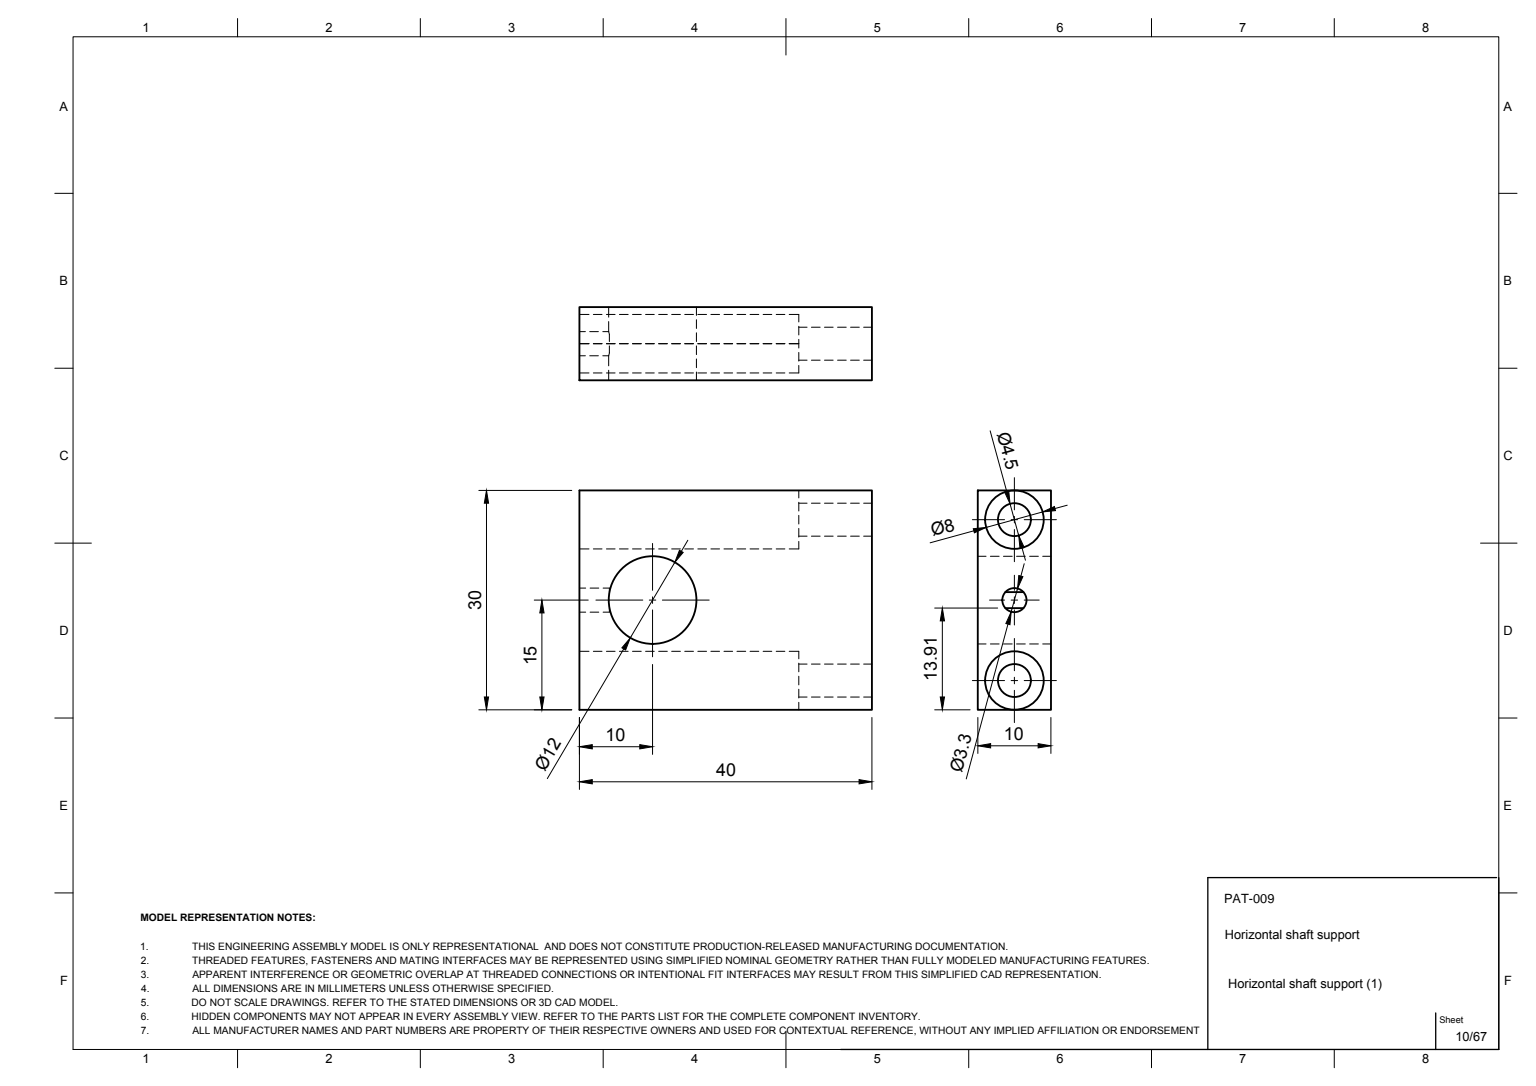
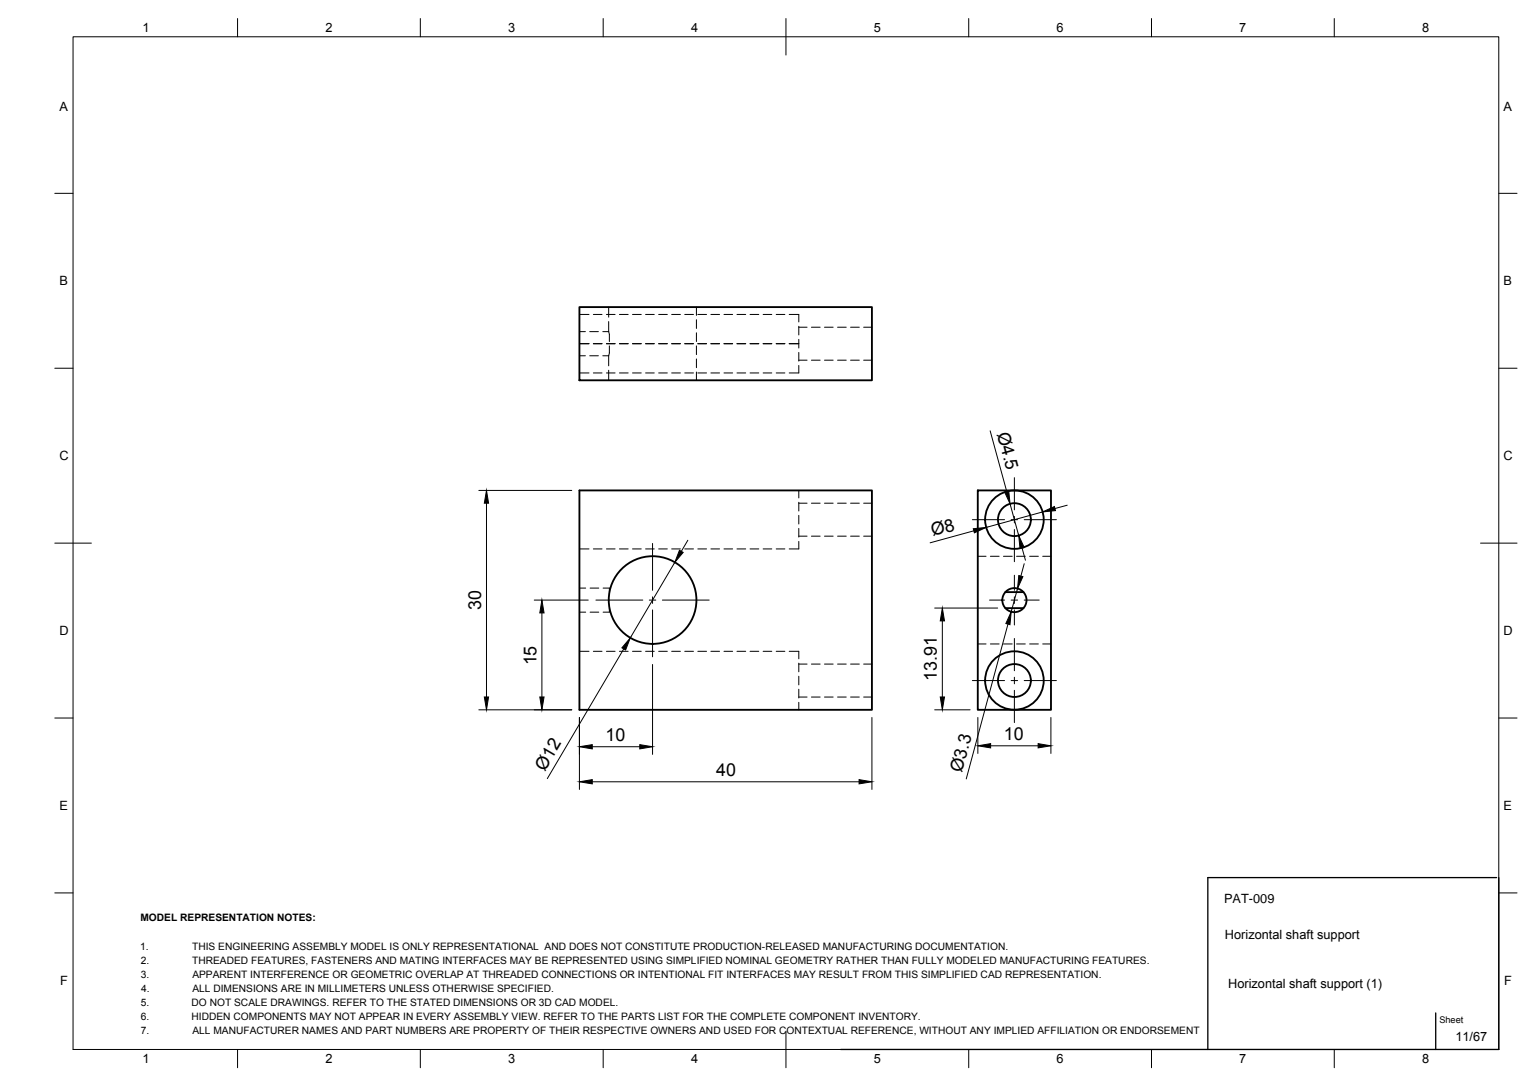
ISO-10303-21;
HEADER;
/* Generated by software containing ST-Developer
 * from STEP Tools, Inc. (www.steptools.com) 
 */

FILE_DESCRIPTION(
/* description */ ('Bell-crank linkage with push rods'),
/* implementation_level */ '2;1');

FILE_NAME(
/* name */ 'Horizontal shaft support (1).step',
/* time_stamp */ '2026-10-28T03:25:15-07:00',
/* author */ (''),
/* organization */ (''),
/* preprocessor_version */ 'ST-DEVELOPER v20.2',
/* originating_system */ 'Autodesk Translation Framework v15.17.0.0',
/* authorisation */ '');

FILE_SCHEMA (('AUTOMOTIVE_DESIGN { 1 0 10303 214 3 1 1 }'));
ENDSEC;

DATA;
#10=MECHANICAL_DESIGN_GEOMETRIC_PRESENTATION_REPRESENTATION('',(#610),#16678);
#465=B_SPLINE_CURVE_WITH_KNOTS('',3,(#14110,#14111,#14112,#14113,#14114,
#14115),.UNSPECIFIED.,.F.,.F.,(4,2,4),(0.635430324955932,0.687528937234027,
0.750024497760672),.UNSPECIFIED.);
#466=B_SPLINE_CURVE_WITH_KNOTS('',3,(#14119,#14120,#14121,#14122,#14123,
#14124),.UNSPECIFIED.,.F.,.F.,(4,2,4),(0.250008165920224,0.312503726446869,
0.364602338724963),.UNSPECIFIED.);
#467=B_SPLINE_CURVE_WITH_KNOTS('',3,(#14125,#14126,#14127,#14128,#14129,
#14130),.UNSPECIFIED.,.F.,.F.,(4,2,4),(0.135413993115483,0.187512605393579,
0.250008165920224),.UNSPECIFIED.);
#468=B_SPLINE_CURVE_WITH_KNOTS('',3,(#14131,#14132,#14133,#14134,#14135,
#14136),.UNSPECIFIED.,.F.,.F.,(4,2,4),(0.750024497760672,0.812520058287317,
0.864618670565412),.UNSPECIFIED.);
#502=SHAPE_REPRESENTATION_RELATIONSHIP('SRR','None',#16918,#556);
#556=ADVANCED_BREP_SHAPE_REPRESENTATION('',(#672),#16623);
#610=STYLED_ITEM('',(#17291),#672);
#672=MANIFOLD_SOLID_BREP('Body1',#8800);
#789=FACE_BOUND('',#1935,.T.);
#790=FACE_BOUND('',#1938,.T.);
#791=FACE_BOUND('',#1940,.T.);
#792=FACE_BOUND('',#1946,.T.);
#793=FACE_BOUND('',#1949,.T.);
#794=FACE_BOUND('',#1951,.T.);
#795=FACE_BOUND('',#1952,.T.);
#1013=PLANE('',#9667);
#1014=PLANE('',#9672);
#1015=PLANE('',#9676);
#1016=PLANE('',#9681);
#1017=PLANE('',#9683);
#1018=PLANE('',#9691);
#1019=PLANE('',#9692);
#1020=PLANE('',#9693);
#1021=PLANE('',#9694);
#1022=PLANE('',#9695);
#1342=FACE_OUTER_BOUND('',#1928,.T.);
#1343=FACE_OUTER_BOUND('',#1929,.T.);
#1344=FACE_OUTER_BOUND('',#1930,.T.);
#1345=FACE_OUTER_BOUND('',#1931,.T.);
#1346=FACE_OUTER_BOUND('',#1932,.T.);
#1347=FACE_OUTER_BOUND('',#1933,.T.);
#1348=FACE_OUTER_BOUND('',#1934,.T.);
#1349=FACE_OUTER_BOUND('',#1936,.T.);
#1350=FACE_OUTER_BOUND('',#1937,.T.);
#1351=FACE_OUTER_BOUND('',#1939,.T.);
#1352=FACE_OUTER_BOUND('',#1941,.T.);
#1353=FACE_OUTER_BOUND('',#1942,.T.);
#1354=FACE_OUTER_BOUND('',#1943,.T.);
#1355=FACE_OUTER_BOUND('',#1944,.T.);
#1356=FACE_OUTER_BOUND('',#1945,.T.);
#1357=FACE_OUTER_BOUND('',#1947,.T.);
#1358=FACE_OUTER_BOUND('',#1948,.T.);
#1359=FACE_OUTER_BOUND('',#1950,.T.);
#1928=EDGE_LOOP('',(#6347,#6348,#6349,#6350));
#1929=EDGE_LOOP('',(#6351,#6352,#6353,#6354));
#1930=EDGE_LOOP('',(#6355,#6356));
#1931=EDGE_LOOP('',(#6357,#6358,#6359,#6360,#6361,#6362,#6363,#6364,#6365));
#1932=EDGE_LOOP('',(#6366,#6367));
#1933=EDGE_LOOP('',(#6368,#6369,#6370,#6371));
#1934=EDGE_LOOP('',(#6372,#6373));
#1935=EDGE_LOOP('',(#6374));
#1936=EDGE_LOOP('',(#6375,#6376,#6377,#6378));
#1937=EDGE_LOOP('',(#6379,#6380));
#1938=EDGE_LOOP('',(#6381));
#1939=EDGE_LOOP('',(#6382,#6383,#6384,#6385,#6386,#6387,#6388,#6389,#6390,
#6391));
#1940=EDGE_LOOP('',(#6392));
#1941=EDGE_LOOP('',(#6393,#6394,#6395,#6396));
#1942=EDGE_LOOP('',(#6397,#6398,#6399,#6400));
#1943=EDGE_LOOP('',(#6401,#6402,#6403,#6404,#6405,#6406,#6407,#6408,#6409,
#6410,#6411,#6412));
#1944=EDGE_LOOP('',(#6413,#6414,#6415,#6416,#6417,#6418,#6419));
#1945=EDGE_LOOP('',(#6420,#6421,#6422,#6423));
#1946=EDGE_LOOP('',(#6424));
#1947=EDGE_LOOP('',(#6425,#6426,#6427,#6428,#6429,#6430,#6431));
#1948=EDGE_LOOP('',(#6432,#6433,#6434,#6435));
#1949=EDGE_LOOP('',(#6436));
#1950=EDGE_LOOP('',(#6437,#6438,#6439,#6440));
#1951=EDGE_LOOP('',(#6441));
#1952=EDGE_LOOP('',(#6442));
#2639=LINE('',#14087,#3188);
#2640=LINE('',#14091,#3189);
#2641=LINE('',#14096,#3190);
#2642=LINE('',#14100,#3191);
#2643=LINE('',#14105,#3192);
#2644=LINE('',#14138,#3193);
#2645=LINE('',#14141,#3194);
#2646=LINE('',#14144,#3195);
#2647=LINE('',#14151,#3196);
#2648=LINE('',#14159,#3197);
#2649=LINE('',#14160,#3198);
#2650=LINE('',#14162,#3199);
#2651=LINE('',#14164,#3200);
#2652=LINE('',#14165,#3201);
#2653=LINE('',#14166,#3202);
#2654=LINE('',#14170,#3203);
#2655=LINE('',#14174,#3204);
#2656=LINE('',#14178,#3205);
#2657=LINE('',#14180,#3206);
#2658=LINE('',#14185,#3207);
#2659=LINE('',#14186,#3208);
#2660=LINE('',#14187,#3209);
#2661=LINE('',#14190,#3210);
#2662=LINE('',#14191,#3211);
#2663=LINE('',#14194,#3212);
#2664=LINE('',#14195,#3213);
#2665=LINE('',#14197,#3214);
#3188=VECTOR('',#11153,0.4);
#3189=VECTOR('',#11156,1.);
#3190=VECTOR('',#11161,0.4);
#3191=VECTOR('',#11164,1.);
#3192=VECTOR('',#11169,1.);
#3193=VECTOR('',#11176,0.164999999999999);
#3194=VECTOR('',#11181,1.);
#3195=VECTOR('',#11186,1.);
#3196=VECTOR('',#11197,1.);
#3197=VECTOR('',#11206,1.);
#3198=VECTOR('',#11207,1.);
#3199=VECTOR('',#11208,1.);
#3200=VECTOR('',#11209,1.);
#3201=VECTOR('',#11210,1.);
#3202=VECTOR('',#11211,1.);
#3203=VECTOR('',#11216,0.225);
#3204=VECTOR('',#11221,0.225);
#3205=VECTOR('',#11226,0.6);
#3206=VECTOR('',#11227,0.6);
#3207=VECTOR('',#11232,1.);
#3208=VECTOR('',#11233,1.);
#3209=VECTOR('',#11234,1.);
#3210=VECTOR('',#11237,1.);
#3211=VECTOR('',#11238,1.);
#3212=VECTOR('',#11241,1.);
#3213=VECTOR('',#11242,1.);
#3214=VECTOR('',#11245,1.);
#3733=CIRCLE('',#9662,0.4);
#3734=CIRCLE('',#9663,0.4);
#3735=CIRCLE('',#9665,0.4);
#3736=CIRCLE('',#9666,0.4);
#3737=CIRCLE('',#9668,0.164999999999999);
#3738=CIRCLE('',#9670,0.164999999999999);
#3739=CIRCLE('',#9671,0.164999999999999);
#3740=CIRCLE('',#9674,0.4);
#3741=CIRCLE('',#9675,0.4);
#3742=CIRCLE('',#9677,0.225);
#3743=CIRCLE('',#9679,0.4);
#3744=CIRCLE('',#9680,0.4);
#3745=CIRCLE('',#9682,0.225);
#3746=CIRCLE('',#9685,0.225);
#3747=CIRCLE('',#9687,0.225);
#3748=CIRCLE('',#9689,0.6);
#3749=CIRCLE('',#9690,0.6);
#4263=VERTEX_POINT('',#14085);
#4264=VERTEX_POINT('',#14086);
#4265=VERTEX_POINT('',#14088);
#4266=VERTEX_POINT('',#14090);
#4267=VERTEX_POINT('',#14094);
#4268=VERTEX_POINT('',#14095);
#4269=VERTEX_POINT('',#14097);
#4270=VERTEX_POINT('',#14099);
#4271=VERTEX_POINT('',#14103);
#4272=VERTEX_POINT('',#14104);
#4273=VERTEX_POINT('',#14108);
#4274=VERTEX_POINT('',#14109);
#4275=VERTEX_POINT('',#14116);
#4276=VERTEX_POINT('',#14118);
#4277=VERTEX_POINT('',#14137);
#4278=VERTEX_POINT('',#14147);
#4279=VERTEX_POINT('',#14154);
#4280=VERTEX_POINT('',#14157);
#4281=VERTEX_POINT('',#14158);
#4282=VERTEX_POINT('',#14161);
#4283=VERTEX_POINT('',#14163);
#4284=VERTEX_POINT('',#14168);
#4285=VERTEX_POINT('',#14172);
#4286=VERTEX_POINT('',#14176);
#4287=VERTEX_POINT('',#14179);
#4288=VERTEX_POINT('',#14183);
#4289=VERTEX_POINT('',#14184);
#4290=VERTEX_POINT('',#14189);
#4291=VERTEX_POINT('',#14193);
#5051=EDGE_CURVE('',#4263,#4264,#2639,.T.);
#5052=EDGE_CURVE('',#4265,#4263,#3733,.T.);
#5053=EDGE_CURVE('',#4265,#4266,#2640,.T.);
#5054=EDGE_CURVE('',#4264,#4266,#3734,.T.);
#5055=EDGE_CURVE('',#4267,#4268,#2641,.T.);
#5056=EDGE_CURVE('',#4269,#4267,#3735,.T.);
#5057=EDGE_CURVE('',#4269,#4270,#2642,.T.);
#5058=EDGE_CURVE('',#4268,#4270,#3736,.T.);
#5059=EDGE_CURVE('',#4271,#4272,#2643,.T.);
#5060=EDGE_CURVE('',#4271,#4272,#3737,.T.);
#5061=EDGE_CURVE('',#4273,#4274,#465,.T.);
#5062=EDGE_CURVE('',#4275,#4273,#3738,.T.);
#5063=EDGE_CURVE('',#4276,#4275,#466,.T.);
#5064=EDGE_CURVE('',#4272,#4276,#467,.T.);
#5065=EDGE_CURVE('',#4274,#4271,#468,.T.);
#5066=EDGE_CURVE('',#4274,#4277,#2644,.T.);
#5067=EDGE_CURVE('',#4277,#4277,#3739,.T.);
#5068=EDGE_CURVE('',#4275,#4273,#2645,.T.);
#5069=EDGE_CURVE('',#4270,#4268,#3740,.T.);
#5070=EDGE_CURVE('',#4269,#4270,#2646,.T.);
#5071=EDGE_CURVE('',#4267,#4269,#3741,.T.);
#5072=EDGE_CURVE('',#4278,#4278,#3742,.T.);
#5073=EDGE_CURVE('',#4266,#4264,#3743,.T.);
#5074=EDGE_CURVE('',#4265,#4266,#2647,.T.);
#5075=EDGE_CURVE('',#4263,#4265,#3744,.T.);
#5076=EDGE_CURVE('',#4279,#4279,#3745,.T.);
#5077=EDGE_CURVE('',#4280,#4281,#2648,.T.);
#5078=EDGE_CURVE('',#4281,#4270,#2649,.T.);
#5079=EDGE_CURVE('',#4270,#4282,#2650,.T.);
#5080=EDGE_CURVE('',#4282,#4283,#2651,.T.);
#5081=EDGE_CURVE('',#4283,#4266,#2652,.T.);
#5082=EDGE_CURVE('',#4266,#4280,#2653,.T.);
#5083=EDGE_CURVE('',#4284,#4284,#3746,.T.);
#5084=EDGE_CURVE('',#4284,#4278,#2654,.T.);
#5085=EDGE_CURVE('',#4285,#4285,#3747,.T.);
#5086=EDGE_CURVE('',#4285,#4279,#2655,.T.);
#5087=EDGE_CURVE('',#4286,#4286,#3748,.T.);
#5088=EDGE_CURVE('',#4286,#4274,#2656,.T.);
#5089=EDGE_CURVE('',#4276,#4287,#2657,.T.);
#5090=EDGE_CURVE('',#4287,#4287,#3749,.T.);
#5091=EDGE_CURVE('',#4288,#4289,#2658,.T.);
#5092=EDGE_CURVE('',#4289,#4280,#2659,.T.);
#5093=EDGE_CURVE('',#4288,#4283,#2660,.T.);
#5094=EDGE_CURVE('',#4290,#4288,#2661,.T.);
#5095=EDGE_CURVE('',#4290,#4282,#2662,.T.);
#5096=EDGE_CURVE('',#4291,#4290,#2663,.T.);
#5097=EDGE_CURVE('',#4291,#4281,#2664,.T.);
#5098=EDGE_CURVE('',#4289,#4291,#2665,.T.);
#6347=ORIENTED_EDGE('',*,*,#5051,.F.);
#6348=ORIENTED_EDGE('',*,*,#5052,.F.);
#6349=ORIENTED_EDGE('',*,*,#5053,.T.);
#6350=ORIENTED_EDGE('',*,*,#5054,.F.);
#6351=ORIENTED_EDGE('',*,*,#5055,.F.);
#6352=ORIENTED_EDGE('',*,*,#5056,.F.);
#6353=ORIENTED_EDGE('',*,*,#5057,.T.);
#6354=ORIENTED_EDGE('',*,*,#5058,.F.);
#6355=ORIENTED_EDGE('',*,*,#5059,.F.);
#6356=ORIENTED_EDGE('',*,*,#5060,.T.);
#6357=ORIENTED_EDGE('',*,*,#5061,.F.);
#6358=ORIENTED_EDGE('',*,*,#5062,.F.);
#6359=ORIENTED_EDGE('',*,*,#5063,.F.);
#6360=ORIENTED_EDGE('',*,*,#5064,.F.);
#6361=ORIENTED_EDGE('',*,*,#5060,.F.);
#6362=ORIENTED_EDGE('',*,*,#5065,.F.);
#6363=ORIENTED_EDGE('',*,*,#5066,.T.);
#6364=ORIENTED_EDGE('',*,*,#5067,.F.);
#6365=ORIENTED_EDGE('',*,*,#5066,.F.);
#6366=ORIENTED_EDGE('',*,*,#5068,.F.);
#6367=ORIENTED_EDGE('',*,*,#5062,.T.);
#6368=ORIENTED_EDGE('',*,*,#5055,.T.);
#6369=ORIENTED_EDGE('',*,*,#5069,.F.);
#6370=ORIENTED_EDGE('',*,*,#5070,.F.);
#6371=ORIENTED_EDGE('',*,*,#5071,.F.);
#6372=ORIENTED_EDGE('',*,*,#5056,.T.);
#6373=ORIENTED_EDGE('',*,*,#5071,.T.);
#6374=ORIENTED_EDGE('',*,*,#5072,.F.);
#6375=ORIENTED_EDGE('',*,*,#5051,.T.);
#6376=ORIENTED_EDGE('',*,*,#5073,.F.);
#6377=ORIENTED_EDGE('',*,*,#5074,.F.);
#6378=ORIENTED_EDGE('',*,*,#5075,.F.);
#6379=ORIENTED_EDGE('',*,*,#5052,.T.);
#6380=ORIENTED_EDGE('',*,*,#5075,.T.);
#6381=ORIENTED_EDGE('',*,*,#5076,.F.);
#6382=ORIENTED_EDGE('',*,*,#5077,.T.);
#6383=ORIENTED_EDGE('',*,*,#5078,.T.);
#6384=ORIENTED_EDGE('',*,*,#5069,.T.);
#6385=ORIENTED_EDGE('',*,*,#5058,.T.);
#6386=ORIENTED_EDGE('',*,*,#5079,.T.);
#6387=ORIENTED_EDGE('',*,*,#5080,.T.);
#6388=ORIENTED_EDGE('',*,*,#5081,.T.);
#6389=ORIENTED_EDGE('',*,*,#5073,.T.);
#6390=ORIENTED_EDGE('',*,*,#5054,.T.);
#6391=ORIENTED_EDGE('',*,*,#5082,.T.);
#6392=ORIENTED_EDGE('',*,*,#5067,.T.);
#6393=ORIENTED_EDGE('',*,*,#5083,.F.);
#6394=ORIENTED_EDGE('',*,*,#5084,.T.);
#6395=ORIENTED_EDGE('',*,*,#5072,.T.);
#6396=ORIENTED_EDGE('',*,*,#5084,.F.);
#6397=ORIENTED_EDGE('',*,*,#5085,.F.);
#6398=ORIENTED_EDGE('',*,*,#5086,.T.);
#6399=ORIENTED_EDGE('',*,*,#5076,.T.);
#6400=ORIENTED_EDGE('',*,*,#5086,.F.);
#6401=ORIENTED_EDGE('',*,*,#5087,.F.);
#6402=ORIENTED_EDGE('',*,*,#5088,.T.);
#6403=ORIENTED_EDGE('',*,*,#5065,.T.);
#6404=ORIENTED_EDGE('',*,*,#5059,.T.);
#6405=ORIENTED_EDGE('',*,*,#5064,.T.);
#6406=ORIENTED_EDGE('',*,*,#5089,.T.);
#6407=ORIENTED_EDGE('',*,*,#5090,.F.);
#6408=ORIENTED_EDGE('',*,*,#5089,.F.);
#6409=ORIENTED_EDGE('',*,*,#5063,.T.);
#6410=ORIENTED_EDGE('',*,*,#5068,.T.);
#6411=ORIENTED_EDGE('',*,*,#5061,.T.);
#6412=ORIENTED_EDGE('',*,*,#5088,.F.);
#6413=ORIENTED_EDGE('',*,*,#5091,.T.);
#6414=ORIENTED_EDGE('',*,*,#5092,.T.);
#6415=ORIENTED_EDGE('',*,*,#5082,.F.);
#6416=ORIENTED_EDGE('',*,*,#5053,.F.);
#6417=ORIENTED_EDGE('',*,*,#5074,.T.);
#6418=ORIENTED_EDGE('',*,*,#5081,.F.);
#6419=ORIENTED_EDGE('',*,*,#5093,.F.);
#6420=ORIENTED_EDGE('',*,*,#5094,.T.);
#6421=ORIENTED_EDGE('',*,*,#5093,.T.);
#6422=ORIENTED_EDGE('',*,*,#5080,.F.);
#6423=ORIENTED_EDGE('',*,*,#5095,.F.);
#6424=ORIENTED_EDGE('',*,*,#5090,.T.);
#6425=ORIENTED_EDGE('',*,*,#5096,.T.);
#6426=ORIENTED_EDGE('',*,*,#5095,.T.);
#6427=ORIENTED_EDGE('',*,*,#5079,.F.);
#6428=ORIENTED_EDGE('',*,*,#5057,.F.);
#6429=ORIENTED_EDGE('',*,*,#5070,.T.);
#6430=ORIENTED_EDGE('',*,*,#5078,.F.);
#6431=ORIENTED_EDGE('',*,*,#5097,.F.);
#6432=ORIENTED_EDGE('',*,*,#5098,.T.);
#6433=ORIENTED_EDGE('',*,*,#5097,.T.);
#6434=ORIENTED_EDGE('',*,*,#5077,.F.);
#6435=ORIENTED_EDGE('',*,*,#5092,.F.);
#6436=ORIENTED_EDGE('',*,*,#5087,.T.);
#6437=ORIENTED_EDGE('',*,*,#5098,.F.);
#6438=ORIENTED_EDGE('',*,*,#5091,.F.);
#6439=ORIENTED_EDGE('',*,*,#5094,.F.);
#6440=ORIENTED_EDGE('',*,*,#5096,.F.);
#6441=ORIENTED_EDGE('',*,*,#5083,.T.);
#6442=ORIENTED_EDGE('',*,*,#5085,.T.);
#8115=CYLINDRICAL_SURFACE('',#9661,0.4);
#8116=CYLINDRICAL_SURFACE('',#9664,0.4);
#8117=CYLINDRICAL_SURFACE('',#9669,0.164999999999999);
#8118=CYLINDRICAL_SURFACE('',#9673,0.4);
#8119=CYLINDRICAL_SURFACE('',#9678,0.4);
#8120=CYLINDRICAL_SURFACE('',#9684,0.225);
#8121=CYLINDRICAL_SURFACE('',#9686,0.225);
#8122=CYLINDRICAL_SURFACE('',#9688,0.6);
#8367=ADVANCED_FACE('',(#1342),#8115,.F.);
#8368=ADVANCED_FACE('',(#1343),#8116,.F.);
#8369=ADVANCED_FACE('',(#1344),#1013,.T.);
#8370=ADVANCED_FACE('',(#1345),#8117,.F.);
#8371=ADVANCED_FACE('',(#1346),#1014,.T.);
#8372=ADVANCED_FACE('',(#1347),#8118,.F.);
#8373=ADVANCED_FACE('',(#1348,#789),#1015,.T.);
#8374=ADVANCED_FACE('',(#1349),#8119,.F.);
#8375=ADVANCED_FACE('',(#1350,#790),#1016,.T.);
#8376=ADVANCED_FACE('',(#1351,#791),#1017,.T.);
#8377=ADVANCED_FACE('',(#1352),#8120,.F.);
#8378=ADVANCED_FACE('',(#1353),#8121,.F.);
#8379=ADVANCED_FACE('',(#1354),#8122,.F.);
#8380=ADVANCED_FACE('',(#1355),#1018,.T.);
#8381=ADVANCED_FACE('',(#1356,#792),#1019,.T.);
#8382=ADVANCED_FACE('',(#1357),#1020,.T.);
#8383=ADVANCED_FACE('',(#1358,#793),#1021,.T.);
#8384=ADVANCED_FACE('',(#1359,#794,#795),#1022,.F.);
#8800=CLOSED_SHELL('',(#8367,#8368,#8369,#8370,#8371,#8372,#8373,#8374,
#8375,#8376,#8377,#8378,#8379,#8380,#8381,#8382,#8383,#8384));
#9660=AXIS2_PLACEMENT_3D('',#14083,#11149,#11150);
#9661=AXIS2_PLACEMENT_3D('',#14084,#11151,#11152);
#9662=AXIS2_PLACEMENT_3D('',#14089,#11154,#11155);
#9663=AXIS2_PLACEMENT_3D('',#14092,#11157,#11158);
#9664=AXIS2_PLACEMENT_3D('',#14093,#11159,#11160);
#9665=AXIS2_PLACEMENT_3D('',#14098,#11162,#11163);
#9666=AXIS2_PLACEMENT_3D('',#14101,#11165,#11166);
#9667=AXIS2_PLACEMENT_3D('',#14102,#11167,#11168);
#9668=AXIS2_PLACEMENT_3D('',#14106,#11170,#11171);
#9669=AXIS2_PLACEMENT_3D('',#14107,#11172,#11173);
#9670=AXIS2_PLACEMENT_3D('',#14117,#11174,#11175);
#9671=AXIS2_PLACEMENT_3D('',#14139,#11177,#11178);
#9672=AXIS2_PLACEMENT_3D('',#14140,#11179,#11180);
#9673=AXIS2_PLACEMENT_3D('',#14142,#11182,#11183);
#9674=AXIS2_PLACEMENT_3D('',#14143,#11184,#11185);
#9675=AXIS2_PLACEMENT_3D('',#14145,#11187,#11188);
#9676=AXIS2_PLACEMENT_3D('',#14146,#11189,#11190);
#9677=AXIS2_PLACEMENT_3D('',#14148,#11191,#11192);
#9678=AXIS2_PLACEMENT_3D('',#14149,#11193,#11194);
#9679=AXIS2_PLACEMENT_3D('',#14150,#11195,#11196);
#9680=AXIS2_PLACEMENT_3D('',#14152,#11198,#11199);
#9681=AXIS2_PLACEMENT_3D('',#14153,#11200,#11201);
#9682=AXIS2_PLACEMENT_3D('',#14155,#11202,#11203);
#9683=AXIS2_PLACEMENT_3D('',#14156,#11204,#11205);
#9684=AXIS2_PLACEMENT_3D('',#14167,#11212,#11213);
#9685=AXIS2_PLACEMENT_3D('',#14169,#11214,#11215);
#9686=AXIS2_PLACEMENT_3D('',#14171,#11217,#11218);
#9687=AXIS2_PLACEMENT_3D('',#14173,#11219,#11220);
#9688=AXIS2_PLACEMENT_3D('',#14175,#11222,#11223);
#9689=AXIS2_PLACEMENT_3D('',#14177,#11224,#11225);
#9690=AXIS2_PLACEMENT_3D('',#14181,#11228,#11229);
#9691=AXIS2_PLACEMENT_3D('',#14182,#11230,#11231);
#9692=AXIS2_PLACEMENT_3D('',#14188,#11235,#11236);
#9693=AXIS2_PLACEMENT_3D('',#14192,#11239,#11240);
#9694=AXIS2_PLACEMENT_3D('',#14196,#11243,#11244);
#9695=AXIS2_PLACEMENT_3D('',#14198,#11246,#11247);
#11149=DIRECTION('axis',(0.,0.,1.));
#11150=DIRECTION('refdir',(1.,0.,0.));
#11151=DIRECTION('center_axis',(0.,0.,1.));
#11152=DIRECTION('ref_axis',(1.,0.,0.));
#11153=DIRECTION('',(0.,0.,1.));
#11154=DIRECTION('center_axis',(0.,0.,1.));
#11155=DIRECTION('ref_axis',(1.,0.,0.));
#11156=DIRECTION('',(0.,0.,1.));
#11157=DIRECTION('center_axis',(0.,0.,-1.));
#11158=DIRECTION('ref_axis',(1.,0.,0.));
#11159=DIRECTION('center_axis',(0.,0.,1.));
#11160=DIRECTION('ref_axis',(1.,0.,0.));
#11161=DIRECTION('',(0.,0.,1.));
#11162=DIRECTION('center_axis',(0.,0.,1.));
#11163=DIRECTION('ref_axis',(1.,0.,0.));
#11164=DIRECTION('',(0.,0.,1.));
#11165=DIRECTION('center_axis',(0.,0.,-1.));
#11166=DIRECTION('ref_axis',(1.,0.,0.));
#11167=DIRECTION('center_axis',(0.,0.,1.));
#11168=DIRECTION('ref_axis',(1.,0.,0.));
#11169=DIRECTION('',(1.,0.,0.));
#11170=DIRECTION('center_axis',(0.,0.,1.));
#11171=DIRECTION('ref_axis',(1.,0.,0.));
#11172=DIRECTION('center_axis',(0.,0.,1.));
#11173=DIRECTION('ref_axis',(1.,0.,0.));
#11174=DIRECTION('center_axis',(0.,0.,1.));
#11175=DIRECTION('ref_axis',(1.,0.,0.));
#11176=DIRECTION('',(0.,0.,1.));
#11177=DIRECTION('center_axis',(0.,0.,-1.));
#11178=DIRECTION('ref_axis',(1.,0.,0.));
#11179=DIRECTION('center_axis',(0.,0.,1.));
#11180=DIRECTION('ref_axis',(1.,0.,0.));
#11181=DIRECTION('',(-1.,0.,0.));
#11182=DIRECTION('center_axis',(0.,0.,1.));
#11183=DIRECTION('ref_axis',(1.,0.,0.));
#11184=DIRECTION('center_axis',(0.,0.,-1.));
#11185=DIRECTION('ref_axis',(1.,0.,0.));
#11186=DIRECTION('',(0.,0.,1.));
#11187=DIRECTION('center_axis',(0.,0.,1.));
#11188=DIRECTION('ref_axis',(1.,0.,0.));
#11189=DIRECTION('center_axis',(0.,0.,1.));
#11190=DIRECTION('ref_axis',(1.,0.,0.));
#11191=DIRECTION('center_axis',(0.,0.,1.));
#11192=DIRECTION('ref_axis',(1.,0.,0.));
#11193=DIRECTION('center_axis',(0.,0.,1.));
#11194=DIRECTION('ref_axis',(1.,0.,0.));
#11195=DIRECTION('center_axis',(0.,0.,-1.));
#11196=DIRECTION('ref_axis',(1.,0.,0.));
#11197=DIRECTION('',(0.,0.,1.));
#11198=DIRECTION('center_axis',(0.,0.,1.));
#11199=DIRECTION('ref_axis',(1.,0.,0.));
#11200=DIRECTION('center_axis',(0.,0.,1.));
#11201=DIRECTION('ref_axis',(1.,0.,0.));
#11202=DIRECTION('center_axis',(0.,0.,1.));
#11203=DIRECTION('ref_axis',(1.,0.,0.));
#11204=DIRECTION('center_axis',(0.,0.,1.));
#11205=DIRECTION('ref_axis',(1.,0.,0.));
#11206=DIRECTION('',(0.,-1.,0.));
#11207=DIRECTION('',(1.,0.,0.));
#11208=DIRECTION('',(1.,0.,0.));
#11209=DIRECTION('',(0.,1.,0.));
#11210=DIRECTION('',(-1.,0.,0.));
#11211=DIRECTION('',(-1.,0.,0.));
#11212=DIRECTION('center_axis',(0.,0.,1.));
#11213=DIRECTION('ref_axis',(1.,0.,0.));
#11214=DIRECTION('center_axis',(0.,0.,1.));
#11215=DIRECTION('ref_axis',(1.,0.,0.));
#11216=DIRECTION('',(0.,0.,1.));
#11217=DIRECTION('center_axis',(0.,0.,1.));
#11218=DIRECTION('ref_axis',(1.,0.,0.));
#11219=DIRECTION('center_axis',(0.,0.,1.));
#11220=DIRECTION('ref_axis',(1.,0.,0.));
#11221=DIRECTION('',(0.,0.,1.));
#11222=DIRECTION('center_axis',(1.,0.,0.));
#11223=DIRECTION('ref_axis',(0.,0.,-1.));
#11224=DIRECTION('center_axis',(1.,0.,0.));
#11225=DIRECTION('ref_axis',(0.,0.,-1.));
#11226=DIRECTION('',(1.,0.,0.));
#11227=DIRECTION('',(1.,0.,0.));
#11228=DIRECTION('center_axis',(-1.,0.,0.));
#11229=DIRECTION('ref_axis',(0.,0.,-1.));
#11230=DIRECTION('center_axis',(0.,1.,0.));
#11231=DIRECTION('ref_axis',(-1.,0.,0.));
#11232=DIRECTION('',(-1.,0.,0.));
#11233=DIRECTION('',(0.,0.,1.));
#11234=DIRECTION('',(0.,0.,1.));
#11235=DIRECTION('center_axis',(1.,0.,0.));
#11236=DIRECTION('ref_axis',(0.,1.,0.));
#11237=DIRECTION('',(0.,1.,0.));
#11238=DIRECTION('',(0.,0.,1.));
#11239=DIRECTION('center_axis',(0.,-1.,0.));
#11240=DIRECTION('ref_axis',(1.,0.,0.));
#11241=DIRECTION('',(1.,0.,0.));
#11242=DIRECTION('',(0.,0.,1.));
#11243=DIRECTION('center_axis',(-1.,0.,0.));
#11244=DIRECTION('ref_axis',(0.,-1.,0.));
#11245=DIRECTION('',(0.,-1.,0.));
#11246=DIRECTION('center_axis',(0.,0.,1.));
#11247=DIRECTION('ref_axis',(1.,0.,0.));
#14083=CARTESIAN_POINT('',(0.,0.,0.));
#14084=CARTESIAN_POINT('Origin',(15.5,3.1,2.));
#14085=CARTESIAN_POINT('',(15.1,3.1,2.));
#14086=CARTESIAN_POINT('',(15.1,3.1,5.));
#14087=CARTESIAN_POINT('',(15.1,3.1,2.));
#14088=CARTESIAN_POINT('',(15.5,3.5,2.));
#14089=CARTESIAN_POINT('Origin',(15.5,3.1,2.));
#14090=CARTESIAN_POINT('',(15.5,3.5,5.));
#14091=CARTESIAN_POINT('',(15.5,3.5,2.));
#14092=CARTESIAN_POINT('Origin',(15.5,3.1,5.));
#14093=CARTESIAN_POINT('Origin',(15.5,0.9,2.));
#14094=CARTESIAN_POINT('',(15.1,0.9,2.));
#14095=CARTESIAN_POINT('',(15.1,0.9,5.));
#14096=CARTESIAN_POINT('',(15.1,0.9,2.));
#14097=CARTESIAN_POINT('',(15.5,0.5,2.));
#14098=CARTESIAN_POINT('Origin',(15.5,0.9,2.));
#14099=CARTESIAN_POINT('',(15.5,0.5,5.));
#14100=CARTESIAN_POINT('',(15.5,0.5,2.));
#14101=CARTESIAN_POINT('Origin',(15.5,0.9,5.));
#14102=CARTESIAN_POINT('Origin',(15.5,2.,4.59));
#14103=CARTESIAN_POINT('',(15.3762058159686,1.89091287885364,4.59));
#14104=CARTESIAN_POINT('',(15.6237941840314,1.89091287885364,4.59));
#14105=CARTESIAN_POINT('',(14.9,1.89091287885364,4.59));
#14106=CARTESIAN_POINT('Origin',(15.5,2.,4.59));
#14107=CARTESIAN_POINT('Origin',(15.5,2.,4.59));
#14108=CARTESIAN_POINT('',(15.3762058159686,2.10908712114636,4.59));
#14109=CARTESIAN_POINT('',(15.335,2.,4.6));
#14110=CARTESIAN_POINT('Ctrl Pts',(15.3762058159686,2.10908712114636,4.59));
#14111=CARTESIAN_POINT('Ctrl Pts',(15.3646008648105,2.09591759715261,4.59243495840567));
#14112=CARTESIAN_POINT('Ctrl Pts',(15.3546543563418,2.08022344943772,4.59485638705045));
#14113=CARTESIAN_POINT('Ctrl Pts',(15.339185135366,2.04298016596019,4.59880705606552));
#14114=CARTESIAN_POINT('Ctrl Pts',(15.335,2.02083185350888,4.6));
#14115=CARTESIAN_POINT('Ctrl Pts',(15.335,2.,4.6));
#14116=CARTESIAN_POINT('',(15.6237941840314,2.10908712114636,4.59));
#14117=CARTESIAN_POINT('Origin',(15.5,2.,4.59));
#14118=CARTESIAN_POINT('',(15.665,2.,4.6));
#14119=CARTESIAN_POINT('Ctrl Pts',(15.665,2.,4.6));
#14120=CARTESIAN_POINT('Ctrl Pts',(15.665,2.02083185350888,4.6));
#14121=CARTESIAN_POINT('Ctrl Pts',(15.660814864634,2.04298016596019,4.59880705606552));
#14122=CARTESIAN_POINT('Ctrl Pts',(15.6453456436582,2.08022344943772,4.59485638705045));
#14123=CARTESIAN_POINT('Ctrl Pts',(15.6353991351895,2.09591759715261,4.59243495840567));
#14124=CARTESIAN_POINT('Ctrl Pts',(15.6237941840314,2.10908712114636,4.59));
#14125=CARTESIAN_POINT('Ctrl Pts',(15.6237941840314,1.89091287885364,4.59));
#14126=CARTESIAN_POINT('Ctrl Pts',(15.6353991351895,1.90408240284739,4.59243495840567));
#14127=CARTESIAN_POINT('Ctrl Pts',(15.6453456436582,1.91977655056228,4.59485638705045));
#14128=CARTESIAN_POINT('Ctrl Pts',(15.660814864634,1.95701983403981,4.59880705606552));
#14129=CARTESIAN_POINT('Ctrl Pts',(15.665,1.97916814649112,4.6));
#14130=CARTESIAN_POINT('Ctrl Pts',(15.665,2.,4.6));
#14131=CARTESIAN_POINT('Ctrl Pts',(15.335,2.,4.6));
#14132=CARTESIAN_POINT('Ctrl Pts',(15.335,1.97916814649112,4.6));
#14133=CARTESIAN_POINT('Ctrl Pts',(15.339185135366,1.95701983403981,4.59880705606552));
#14134=CARTESIAN_POINT('Ctrl Pts',(15.3546543563418,1.91977655056228,4.59485638705045));
#14135=CARTESIAN_POINT('Ctrl Pts',(15.3646008648105,1.90408240284739,4.59243495840567));
#14136=CARTESIAN_POINT('Ctrl Pts',(15.3762058159686,1.89091287885364,4.59));
#14137=CARTESIAN_POINT('',(15.335,2.,5.));
#14138=CARTESIAN_POINT('',(15.335,2.,4.59));
#14139=CARTESIAN_POINT('Origin',(15.5,2.,5.));
#14140=CARTESIAN_POINT('Origin',(15.5,2.,4.59));
#14141=CARTESIAN_POINT('',(14.9,2.10908712114636,4.59));
#14142=CARTESIAN_POINT('Origin',(15.5,0.9,2.));
#14143=CARTESIAN_POINT('Origin',(15.5,0.9,5.));
#14144=CARTESIAN_POINT('',(15.5,0.5,2.));
#14145=CARTESIAN_POINT('Origin',(15.5,0.9,2.));
#14146=CARTESIAN_POINT('Origin',(15.5,0.9,2.));
#14147=CARTESIAN_POINT('',(15.275,0.9,2.));
#14148=CARTESIAN_POINT('Origin',(15.5,0.9,2.));
#14149=CARTESIAN_POINT('Origin',(15.5,3.1,2.));
#14150=CARTESIAN_POINT('Origin',(15.5,3.1,5.));
#14151=CARTESIAN_POINT('',(15.5,3.5,2.));
#14152=CARTESIAN_POINT('Origin',(15.5,3.1,2.));
#14153=CARTESIAN_POINT('Origin',(15.5,3.1,2.));
#14154=CARTESIAN_POINT('',(15.275,3.1,2.));
#14155=CARTESIAN_POINT('Origin',(15.5,3.1,2.));
#14156=CARTESIAN_POINT('Origin',(15.5,2.,5.));
#14157=CARTESIAN_POINT('',(15.,3.5,5.));
#14158=CARTESIAN_POINT('',(15.,0.5,5.));
#14159=CARTESIAN_POINT('',(15.,3.5,5.));
#14160=CARTESIAN_POINT('',(15.,0.5,5.));
#14161=CARTESIAN_POINT('',(16.,0.5,5.));
#14162=CARTESIAN_POINT('',(15.,0.5,5.));
#14163=CARTESIAN_POINT('',(16.,3.5,5.));
#14164=CARTESIAN_POINT('',(16.,0.5,5.));
#14165=CARTESIAN_POINT('',(16.,3.5,5.));
#14166=CARTESIAN_POINT('',(16.,3.5,5.));
#14167=CARTESIAN_POINT('Origin',(15.5,0.9,0.9));
#14168=CARTESIAN_POINT('',(15.275,0.9,1.));
#14169=CARTESIAN_POINT('Origin',(15.5,0.9,1.));
#14170=CARTESIAN_POINT('',(15.275,0.9,0.9));
#14171=CARTESIAN_POINT('Origin',(15.5,3.1,0.9));
#14172=CARTESIAN_POINT('',(15.275,3.1,1.));
#14173=CARTESIAN_POINT('Origin',(15.5,3.1,1.));
#14174=CARTESIAN_POINT('',(15.275,3.1,0.9));
#14175=CARTESIAN_POINT('Origin',(14.9,2.,4.));
#14176=CARTESIAN_POINT('',(15.,2.,4.6));
#14177=CARTESIAN_POINT('Origin',(15.,2.,4.));
#14178=CARTESIAN_POINT('',(14.9,2.,4.6));
#14179=CARTESIAN_POINT('',(16.,2.,4.6));
#14180=CARTESIAN_POINT('',(14.9,2.,4.6));
#14181=CARTESIAN_POINT('Origin',(16.,2.,4.));
#14182=CARTESIAN_POINT('Origin',(16.,3.5,1.));
#14183=CARTESIAN_POINT('',(16.,3.5,1.));
#14184=CARTESIAN_POINT('',(15.,3.5,1.));
#14185=CARTESIAN_POINT('',(16.,3.5,1.));
#14186=CARTESIAN_POINT('',(15.,3.5,1.));
#14187=CARTESIAN_POINT('',(16.,3.5,1.));
#14188=CARTESIAN_POINT('Origin',(16.,0.5,1.));
#14189=CARTESIAN_POINT('',(16.,0.5,1.));
#14190=CARTESIAN_POINT('',(16.,0.5,1.));
#14191=CARTESIAN_POINT('',(16.,0.5,1.));
#14192=CARTESIAN_POINT('Origin',(15.,0.5,1.));
#14193=CARTESIAN_POINT('',(15.,0.5,1.));
#14194=CARTESIAN_POINT('',(15.,0.5,1.));
#14195=CARTESIAN_POINT('',(15.,0.5,1.));
#14196=CARTESIAN_POINT('Origin',(15.,3.5,1.));
#14197=CARTESIAN_POINT('',(15.,3.5,1.));
#14198=CARTESIAN_POINT('Origin',(15.5,2.,1.));
#16559=UNCERTAINTY_MEASURE_WITH_UNIT(LENGTH_MEASURE(0.001),#16679,
'DISTANCE_ACCURACY_VALUE',
'Maximum model space distance between geometric entities at asserted c
onnectivities');
#16614=UNCERTAINTY_MEASURE_WITH_UNIT(LENGTH_MEASURE(0.001),#16679,
'DISTANCE_ACCURACY_VALUE',
'Maximum model space distance between geometric entities at asserted c
onnectivities');
#16623=(
GEOMETRIC_REPRESENTATION_CONTEXT(3)
GLOBAL_UNCERTAINTY_ASSIGNED_CONTEXT((#16559))
GLOBAL_UNIT_ASSIGNED_CONTEXT((#16679,#16681,#16682))
REPRESENTATION_CONTEXT('','3D')
);
#16678=(
GEOMETRIC_REPRESENTATION_CONTEXT(3)
GLOBAL_UNCERTAINTY_ASSIGNED_CONTEXT((#16614))
GLOBAL_UNIT_ASSIGNED_CONTEXT((#16679,#16681,#16682))
REPRESENTATION_CONTEXT('','3D')
);
#16679=(
LENGTH_UNIT()
NAMED_UNIT(*)
SI_UNIT(.CENTI.,.METRE.)
);
#16681=(
NAMED_UNIT(*)
PLANE_ANGLE_UNIT()
SI_UNIT($,.RADIAN.)
);
#16682=(
NAMED_UNIT(*)
SI_UNIT($,.STERADIAN.)
SOLID_ANGLE_UNIT()
);
#16691=SHAPE_DEFINITION_REPRESENTATION(#16754,#16918);
#16754=PRODUCT_DEFINITION_SHAPE('',$,#16982);
#16918=SHAPE_REPRESENTATION('',(#9660),#16623);
#16973=PRODUCT_DEFINITION_CONTEXT('part definition',#17164,'design');
#16982=PRODUCT_DEFINITION('Horizontal shaft support (1)',
'Horizontal shaft support (1)',#17045,#16973);
#17045=PRODUCT_DEFINITION_FORMATION('',$,#17174);
#17164=APPLICATION_CONTEXT(
'Core Data for Automotive Mechanical Design Process');
#17165=PRODUCT_CONTEXT('part definition',#17164,'mechanical');
#17174=PRODUCT('Horizontal shaft support (1)',
'Horizontal shaft support (1)','Horizontal shaft support (1)',(#17165));
#17285=COLOUR_RGB('Grey',0.48,0.52,0.57);
#17286=FILL_AREA_STYLE_COLOUR('',#17285);
#17287=FILL_AREA_STYLE('',(#17286));
#17288=SURFACE_STYLE_FILL_AREA(#17287);
#17289=SURFACE_SIDE_STYLE('',(#17288));
#17290=SURFACE_STYLE_USAGE(.BOTH.,#17289);
#17291=PRESENTATION_STYLE_ASSIGNMENT((#17290));
ENDSEC;
END-ISO-10303-21;
